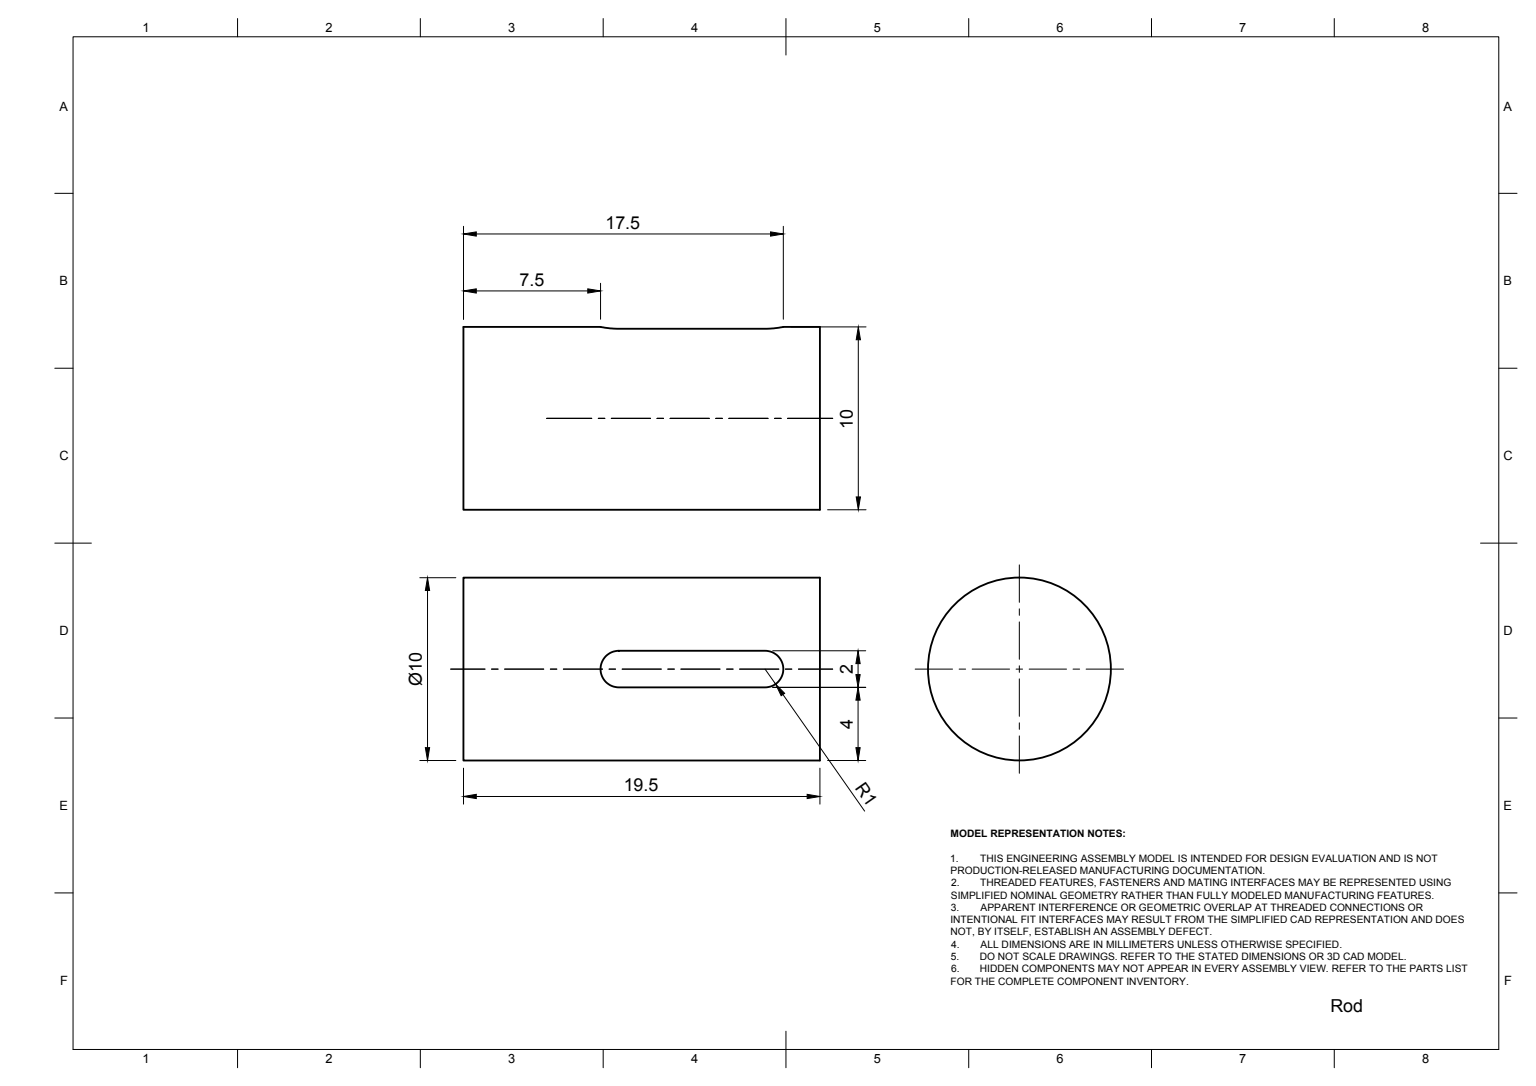
ISO-10303-21;
HEADER;
/* Generated by software containing ST-Developer
 * from STEP Tools, Inc. (www.steptools.com) 
 */

FILE_DESCRIPTION(
/* description */ (''),
/* implementation_level */ '2;1');

FILE_NAME(
/* name */ 'Rod.step',
/* time_stamp */ '2026-10-05T21:34:53-07:00',
/* author */ (''),
/* organization */ (''),
/* preprocessor_version */ 'ST-DEVELOPER v20.2',
/* originating_system */ 'Autodesk Translation Framework v15.15.0.0',
/* authorisation */ '');

FILE_SCHEMA (('AUTOMOTIVE_DESIGN { 1 0 10303 214 3 1 1 }'));
ENDSEC;

DATA;
#10=MECHANICAL_DESIGN_GEOMETRIC_PRESENTATION_REPRESENTATION('',(#70),#9822);
#52=SHAPE_REPRESENTATION_RELATIONSHIP('SRR','None',#9862,#61);
#61=ADVANCED_BREP_SHAPE_REPRESENTATION('',(#79),#9818);
#70=STYLED_ITEM('',(#9912),#79);
#79=MANIFOLD_SOLID_BREP('Body1',#3293);
#97=FACE_BOUND('',#628,.T.);
#153=B_SPLINE_CURVE_WITH_KNOTS('',3,(#9614,#9615,#9616,#9617,#9618,#9619,
#9620,#9621,#9622,#9623,#9624,#9625,#9626,#9627,#9628,#9629,#9630,#9631),
 .UNSPECIFIED.,.F.,.F.,(4,2,2,2,2,2,2,2,4),(0.,0.0377795255890194,0.0755590511780388,
0.113336459804459,0.151113868430879,0.188891277057298,0.226668685683718,
0.264448211272738,0.302227736861757),.UNSPECIFIED.);
#154=B_SPLINE_CURVE_WITH_KNOTS('',3,(#9644,#9645,#9646,#9647,#9648,#9649,
#9650,#9651,#9652,#9653,#9654,#9655,#9656,#9657,#9658,#9659,#9660,#9661),
 .UNSPECIFIED.,.F.,.F.,(4,2,2,2,2,2,2,2,4),(0.302227736861757,0.340007262450777,
0.377786788039796,0.415564196666216,0.453341605292636,0.491119013919056,
0.528896422545476,0.566675948134495,0.604455473723515),.UNSPECIFIED.);
#247=PLANE('',#3671);
#248=PLANE('',#3674);
#249=PLANE('',#3676);
#250=PLANE('',#3678);
#251=PLANE('',#3682);
#422=FACE_OUTER_BOUND('',#621,.T.);
#423=FACE_OUTER_BOUND('',#622,.T.);
#424=FACE_OUTER_BOUND('',#623,.T.);
#425=FACE_OUTER_BOUND('',#624,.T.);
#426=FACE_OUTER_BOUND('',#625,.T.);
#427=FACE_OUTER_BOUND('',#626,.T.);
#428=FACE_OUTER_BOUND('',#627,.T.);
#429=FACE_OUTER_BOUND('',#629,.T.);
#621=EDGE_LOOP('',(#2918,#2919,#2920,#2921));
#622=EDGE_LOOP('',(#2922,#2923,#2924,#2925));
#623=EDGE_LOOP('',(#2926,#2927,#2928,#2929));
#624=EDGE_LOOP('',(#2930,#2931,#2932,#2933));
#625=EDGE_LOOP('',(#2934,#2935,#2936,#2937));
#626=EDGE_LOOP('',(#2938));
#627=EDGE_LOOP('',(#2939,#2940,#2941,#2942));
#628=EDGE_LOOP('',(#2943,#2944,#2945,#2946));
#629=EDGE_LOOP('',(#2947));
#876=LINE('',#9606,#1135);
#877=LINE('',#9608,#1136);
#878=LINE('',#9610,#1137);
#879=LINE('',#9611,#1138);
#880=LINE('',#9634,#1139);
#881=LINE('',#9638,#1140);
#882=LINE('',#9641,#1141);
#883=LINE('',#9642,#1142);
#884=LINE('',#9668,#1143);
#1135=VECTOR('',#4502,10.);
#1136=VECTOR('',#4503,10.);
#1137=VECTOR('',#4504,10.);
#1138=VECTOR('',#4505,10.);
#1139=VECTOR('',#4510,10.);
#1140=VECTOR('',#4515,10.);
#1141=VECTOR('',#4518,10.);
#1142=VECTOR('',#4519,10.);
#1143=VECTOR('',#4530,5.);
#1303=CIRCLE('',#3673,1.);
#1304=CIRCLE('',#3675,1.);
#1305=CIRCLE('',#3679,5.);
#1306=CIRCLE('',#3681,5.);
#1589=VERTEX_POINT('',#9604);
#1590=VERTEX_POINT('',#9605);
#1591=VERTEX_POINT('',#9607);
#1592=VERTEX_POINT('',#9609);
#1593=VERTEX_POINT('',#9613);
#1594=VERTEX_POINT('',#9632);
#1595=VERTEX_POINT('',#9636);
#1596=VERTEX_POINT('',#9640);
#1597=VERTEX_POINT('',#9663);
#1598=VERTEX_POINT('',#9666);
#2038=EDGE_CURVE('',#1589,#1590,#876,.T.);
#2039=EDGE_CURVE('',#1591,#1589,#877,.T.);
#2040=EDGE_CURVE('',#1592,#1591,#878,.T.);
#2041=EDGE_CURVE('',#1592,#1590,#879,.T.);
#2042=EDGE_CURVE('',#1590,#1593,#153,.T.);
#2043=EDGE_CURVE('',#1594,#1592,#1303,.T.);
#2044=EDGE_CURVE('',#1594,#1593,#880,.T.);
#2045=EDGE_CURVE('',#1591,#1595,#1304,.T.);
#2046=EDGE_CURVE('',#1595,#1594,#881,.T.);
#2047=EDGE_CURVE('',#1593,#1596,#882,.T.);
#2048=EDGE_CURVE('',#1595,#1596,#883,.T.);
#2049=EDGE_CURVE('',#1596,#1589,#154,.T.);
#2050=EDGE_CURVE('',#1597,#1597,#1305,.T.);
#2051=EDGE_CURVE('',#1598,#1598,#1306,.T.);
#2052=EDGE_CURVE('',#1598,#1597,#884,.T.);
#2918=ORIENTED_EDGE('',*,*,#2038,.F.);
#2919=ORIENTED_EDGE('',*,*,#2039,.F.);
#2920=ORIENTED_EDGE('',*,*,#2040,.F.);
#2921=ORIENTED_EDGE('',*,*,#2041,.T.);
#2922=ORIENTED_EDGE('',*,*,#2042,.F.);
#2923=ORIENTED_EDGE('',*,*,#2041,.F.);
#2924=ORIENTED_EDGE('',*,*,#2043,.F.);
#2925=ORIENTED_EDGE('',*,*,#2044,.T.);
#2926=ORIENTED_EDGE('',*,*,#2043,.T.);
#2927=ORIENTED_EDGE('',*,*,#2040,.T.);
#2928=ORIENTED_EDGE('',*,*,#2045,.T.);
#2929=ORIENTED_EDGE('',*,*,#2046,.T.);
#2930=ORIENTED_EDGE('',*,*,#2047,.F.);
#2931=ORIENTED_EDGE('',*,*,#2044,.F.);
#2932=ORIENTED_EDGE('',*,*,#2046,.F.);
#2933=ORIENTED_EDGE('',*,*,#2048,.T.);
#2934=ORIENTED_EDGE('',*,*,#2049,.F.);
#2935=ORIENTED_EDGE('',*,*,#2048,.F.);
#2936=ORIENTED_EDGE('',*,*,#2045,.F.);
#2937=ORIENTED_EDGE('',*,*,#2039,.T.);
#2938=ORIENTED_EDGE('',*,*,#2050,.T.);
#2939=ORIENTED_EDGE('',*,*,#2051,.F.);
#2940=ORIENTED_EDGE('',*,*,#2052,.T.);
#2941=ORIENTED_EDGE('',*,*,#2050,.F.);
#2942=ORIENTED_EDGE('',*,*,#2052,.F.);
#2943=ORIENTED_EDGE('',*,*,#2047,.T.);
#2944=ORIENTED_EDGE('',*,*,#2049,.T.);
#2945=ORIENTED_EDGE('',*,*,#2038,.T.);
#2946=ORIENTED_EDGE('',*,*,#2042,.T.);
#2947=ORIENTED_EDGE('',*,*,#2051,.T.);
#3093=CYLINDRICAL_SURFACE('',#3672,1.);
#3094=CYLINDRICAL_SURFACE('',#3677,1.);
#3095=CYLINDRICAL_SURFACE('',#3680,5.);
#3260=ADVANCED_FACE('',(#422),#247,.F.);
#3261=ADVANCED_FACE('',(#423),#3093,.F.);
#3262=ADVANCED_FACE('',(#424),#248,.F.);
#3263=ADVANCED_FACE('',(#425),#249,.F.);
#3264=ADVANCED_FACE('',(#426),#3094,.F.);
#3265=ADVANCED_FACE('',(#427),#250,.F.);
#3266=ADVANCED_FACE('',(#428,#97),#3095,.T.);
#3267=ADVANCED_FACE('',(#429),#251,.T.);
#3293=CLOSED_SHELL('',(#3260,#3261,#3262,#3263,#3264,#3265,#3266,#3267));
#3670=AXIS2_PLACEMENT_3D('',#9602,#4498,#4499);
#3671=AXIS2_PLACEMENT_3D('',#9603,#4500,#4501);
#3672=AXIS2_PLACEMENT_3D('',#9612,#4506,#4507);
#3673=AXIS2_PLACEMENT_3D('',#9633,#4508,#4509);
#3674=AXIS2_PLACEMENT_3D('',#9635,#4511,#4512);
#3675=AXIS2_PLACEMENT_3D('',#9637,#4513,#4514);
#3676=AXIS2_PLACEMENT_3D('',#9639,#4516,#4517);
#3677=AXIS2_PLACEMENT_3D('',#9643,#4520,#4521);
#3678=AXIS2_PLACEMENT_3D('',#9662,#4522,#4523);
#3679=AXIS2_PLACEMENT_3D('',#9664,#4524,#4525);
#3680=AXIS2_PLACEMENT_3D('',#9665,#4526,#4527);
#3681=AXIS2_PLACEMENT_3D('',#9667,#4528,#4529);
#3682=AXIS2_PLACEMENT_3D('',#9669,#4531,#4532);
#4498=DIRECTION('axis',(0.,0.,1.));
#4499=DIRECTION('refdir',(1.,0.,0.));
#4500=DIRECTION('center_axis',(1.,0.,0.));
#4501=DIRECTION('ref_axis',(0.,0.,1.));
#4502=DIRECTION('',(0.,0.,-1.));
#4503=DIRECTION('',(0.,-1.,0.));
#4504=DIRECTION('',(0.,0.,1.));
#4505=DIRECTION('',(0.,-1.,0.));
#4506=DIRECTION('center_axis',(0.,-1.,0.));
#4507=DIRECTION('ref_axis',(1.,0.,0.));
#4508=DIRECTION('center_axis',(0.,-1.,0.));
#4509=DIRECTION('ref_axis',(1.,0.,0.));
#4510=DIRECTION('',(0.,-1.,0.));
#4511=DIRECTION('center_axis',(0.,1.,0.));
#4512=DIRECTION('ref_axis',(1.,0.,0.));
#4513=DIRECTION('center_axis',(0.,-1.,0.));
#4514=DIRECTION('ref_axis',(-1.,0.,0.));
#4515=DIRECTION('',(0.,0.,-1.));
#4516=DIRECTION('center_axis',(-1.,0.,0.));
#4517=DIRECTION('ref_axis',(0.,0.,-1.));
#4518=DIRECTION('',(0.,0.,1.));
#4519=DIRECTION('',(0.,-1.,0.));
#4520=DIRECTION('center_axis',(0.,-1.,0.));
#4521=DIRECTION('ref_axis',(-1.,0.,0.));
#4522=DIRECTION('center_axis',(0.,0.,1.));
#4523=DIRECTION('ref_axis',(-1.,0.,0.));
#4524=DIRECTION('center_axis',(0.,0.,-1.));
#4525=DIRECTION('ref_axis',(-1.,0.,0.));
#4526=DIRECTION('center_axis',(0.,0.,1.));
#4527=DIRECTION('ref_axis',(-1.,0.,0.));
#4528=DIRECTION('center_axis',(0.,0.,1.));
#4529=DIRECTION('ref_axis',(-1.,0.,0.));
#4530=DIRECTION('',(0.,0.,-1.));
#4531=DIRECTION('center_axis',(0.,0.,1.));
#4532=DIRECTION('ref_axis',(-1.,0.,0.));
#9602=CARTESIAN_POINT('',(0.,0.,0.));
#9603=CARTESIAN_POINT('Origin',(1.,0.,6.5));
#9604=CARTESIAN_POINT('',(1.,-4.89897948556636,14.5));
#9605=CARTESIAN_POINT('',(1.,-4.89897948556636,6.5));
#9606=CARTESIAN_POINT('',(1.,-4.89897948556636,12.));
#9607=CARTESIAN_POINT('',(1.,-4.,14.5));
#9608=CARTESIAN_POINT('',(1.,0.,14.5));
#9609=CARTESIAN_POINT('',(1.,-4.,6.5));
#9610=CARTESIAN_POINT('',(1.,-4.,8.5));
#9611=CARTESIAN_POINT('',(1.,0.,6.5));
#9612=CARTESIAN_POINT('Origin',(0.,0.,6.5));
#9613=CARTESIAN_POINT('',(-1.,-4.89897948556636,6.5));
#9614=CARTESIAN_POINT('Ctrl Pts',(1.,-4.89897948556636,6.5));
#9615=CARTESIAN_POINT('Ctrl Pts',(1.,-4.89897948556636,6.3740682480366));
#9616=CARTESIAN_POINT('Ctrl Pts',(0.974762796248614,-4.90433876618447,6.23998222283811));
#9617=CARTESIAN_POINT('Ctrl Pts',(0.872605417648382,-4.92354150792771,5.99370799496995));
#9618=CARTESIAN_POINT('Ctrl Pts',(0.795703102192088,-4.93709085101933,5.88148953981899));
#9619=CARTESIAN_POINT('Ctrl Pts',(0.618515424645094,-4.96240337638318,5.704301862272));
#9620=CARTESIAN_POINT('Ctrl Pts',(0.506294861197626,-4.97583347151864,5.62739565845524));
#9621=CARTESIAN_POINT('Ctrl Pts',(0.260013306081865,-4.99476188647081,5.52523545776417));
#9622=CARTESIAN_POINT('Ctrl Pts',(0.125924695421399,-5.,5.5));
#9623=CARTESIAN_POINT('Ctrl Pts',(-0.1259246954214,-5.,5.5));
#9624=CARTESIAN_POINT('Ctrl Pts',(-0.260013306081865,-4.99476188647081,
5.52523545776417));
#9625=CARTESIAN_POINT('Ctrl Pts',(-0.506294861197626,-4.97583347151864,
5.62739565845524));
#9626=CARTESIAN_POINT('Ctrl Pts',(-0.618515424645094,-4.96240337638318,
5.704301862272));
#9627=CARTESIAN_POINT('Ctrl Pts',(-0.795703102192089,-4.93709085101933,
5.88148953981899));
#9628=CARTESIAN_POINT('Ctrl Pts',(-0.872605417648384,-4.92354150792771,
5.99370799496995));
#9629=CARTESIAN_POINT('Ctrl Pts',(-0.974762796248615,-4.90433876618447,
6.23998222283811));
#9630=CARTESIAN_POINT('Ctrl Pts',(-1.,-4.89897948556636,6.3740682480366));
#9631=CARTESIAN_POINT('Ctrl Pts',(-1.,-4.89897948556636,6.5));
#9632=CARTESIAN_POINT('',(-1.,-4.,6.5));
#9633=CARTESIAN_POINT('Origin',(0.,-4.,6.5));
#9634=CARTESIAN_POINT('',(-1.,0.,6.5));
#9635=CARTESIAN_POINT('Origin',(0.,-4.,10.5));
#9636=CARTESIAN_POINT('',(-1.,-4.,14.5));
#9637=CARTESIAN_POINT('Origin',(0.,-4.,14.5));
#9638=CARTESIAN_POINT('',(-1.,-4.,12.5));
#9639=CARTESIAN_POINT('Origin',(-1.,0.,14.5));
#9640=CARTESIAN_POINT('',(-1.,-4.89897948556636,14.5));
#9641=CARTESIAN_POINT('',(-1.,-4.89897948556636,12.));
#9642=CARTESIAN_POINT('',(-1.,0.,14.5));
#9643=CARTESIAN_POINT('Origin',(0.,0.,14.5));
#9644=CARTESIAN_POINT('Ctrl Pts',(-1.,-4.89897948556636,14.5));
#9645=CARTESIAN_POINT('Ctrl Pts',(-1.,-4.89897948556636,14.6259317519634));
#9646=CARTESIAN_POINT('Ctrl Pts',(-0.974762796248614,-4.90433876618447,
14.7600177771619));
#9647=CARTESIAN_POINT('Ctrl Pts',(-0.872605417648382,-4.92354150792771,
15.0062920050301));
#9648=CARTESIAN_POINT('Ctrl Pts',(-0.795703102192089,-4.93709085101933,
15.118510460181));
#9649=CARTESIAN_POINT('Ctrl Pts',(-0.618515424645094,-4.96240337638318,
15.295698137728));
#9650=CARTESIAN_POINT('Ctrl Pts',(-0.506294861197627,-4.97583347151864,
15.3726043415448));
#9651=CARTESIAN_POINT('Ctrl Pts',(-0.260013306081865,-4.99476188647081,
15.4747645422358));
#9652=CARTESIAN_POINT('Ctrl Pts',(-0.1259246954214,-5.,15.5));
#9653=CARTESIAN_POINT('Ctrl Pts',(0.125924695421399,-5.,15.5));
#9654=CARTESIAN_POINT('Ctrl Pts',(0.260013306081865,-4.99476188647081,15.4747645422358));
#9655=CARTESIAN_POINT('Ctrl Pts',(0.506294861197627,-4.97583347151864,15.3726043415448));
#9656=CARTESIAN_POINT('Ctrl Pts',(0.618515424645094,-4.96240337638318,15.295698137728));
#9657=CARTESIAN_POINT('Ctrl Pts',(0.795703102192089,-4.93709085101933,15.118510460181));
#9658=CARTESIAN_POINT('Ctrl Pts',(0.872605417648383,-4.92354150792771,15.0062920050301));
#9659=CARTESIAN_POINT('Ctrl Pts',(0.974762796248613,-4.90433876618447,14.7600177771619));
#9660=CARTESIAN_POINT('Ctrl Pts',(1.,-4.89897948556636,14.6259317519634));
#9661=CARTESIAN_POINT('Ctrl Pts',(1.,-4.89897948556636,14.5));
#9662=CARTESIAN_POINT('Origin',(0.,0.,3.5));
#9663=CARTESIAN_POINT('',(5.,6.12323399573677E-16,3.5));
#9664=CARTESIAN_POINT('Origin',(0.,0.,3.5));
#9665=CARTESIAN_POINT('Origin',(0.,0.,12.));
#9666=CARTESIAN_POINT('',(5.,6.12323399573677E-16,23.));
#9667=CARTESIAN_POINT('Origin',(0.,0.,23.));
#9668=CARTESIAN_POINT('',(5.,6.12323399573677E-16,12.));
#9669=CARTESIAN_POINT('Origin',(0.,0.,23.));
#9807=UNCERTAINTY_MEASURE_WITH_UNIT(LENGTH_MEASURE(0.01),#9823,
'DISTANCE_ACCURACY_VALUE',
'Maximum model space distance between geometric entities at asserted c
onnectivities');
#9811=UNCERTAINTY_MEASURE_WITH_UNIT(LENGTH_MEASURE(0.01),#9823,
'DISTANCE_ACCURACY_VALUE',
'Maximum model space distance between geometric entities at asserted c
onnectivities');
#9818=(
GEOMETRIC_REPRESENTATION_CONTEXT(3)
GLOBAL_UNCERTAINTY_ASSIGNED_CONTEXT((#9807))
GLOBAL_UNIT_ASSIGNED_CONTEXT((#9823,#9825,#9826))
REPRESENTATION_CONTEXT('','3D')
);
#9822=(
GEOMETRIC_REPRESENTATION_CONTEXT(3)
GLOBAL_UNCERTAINTY_ASSIGNED_CONTEXT((#9811))
GLOBAL_UNIT_ASSIGNED_CONTEXT((#9823,#9825,#9826))
REPRESENTATION_CONTEXT('','3D')
);
#9823=(
LENGTH_UNIT()
NAMED_UNIT(*)
SI_UNIT(.MILLI.,.METRE.)
);
#9825=(
NAMED_UNIT(*)
PLANE_ANGLE_UNIT()
SI_UNIT($,.RADIAN.)
);
#9826=(
NAMED_UNIT(*)
SI_UNIT($,.STERADIAN.)
SOLID_ANGLE_UNIT()
);
#9833=SHAPE_DEFINITION_REPRESENTATION(#9843,#9862);
#9843=PRODUCT_DEFINITION_SHAPE('',$,#9873);
#9862=SHAPE_REPRESENTATION('',(#3670),#9818);
#9866=PRODUCT_DEFINITION_CONTEXT('part definition',#9898,'design');
#9873=PRODUCT_DEFINITION('Rod','Rod',#9883,#9866);
#9883=PRODUCT_DEFINITION_FORMATION('',$,#9906);
#9898=APPLICATION_CONTEXT(
'Core Data for Automotive Mechanical Design Process');
#9899=PRODUCT_CONTEXT('part definition',#9898,'mechanical');
#9906=PRODUCT('Rod','Rod',$,(#9899));
#9912=PRESENTATION_STYLE_ASSIGNMENT((#9915));
#9915=SURFACE_STYLE_USAGE(.BOTH.,#9918);
#9918=SURFACE_SIDE_STYLE('',(#9921));
#9921=SURFACE_STYLE_FILL_AREA(#9924);
#9924=FILL_AREA_STYLE('Opaque(233,233,233)',(#9927));
#9927=FILL_AREA_STYLE_COLOUR('Opaque(233,233,233)',#9930);
#9930=COLOUR_RGB('Opaque(233,233,233)', 0.40784314, 0.44705882, 0.49803922);
ENDSEC;
END-ISO-10303-21;
